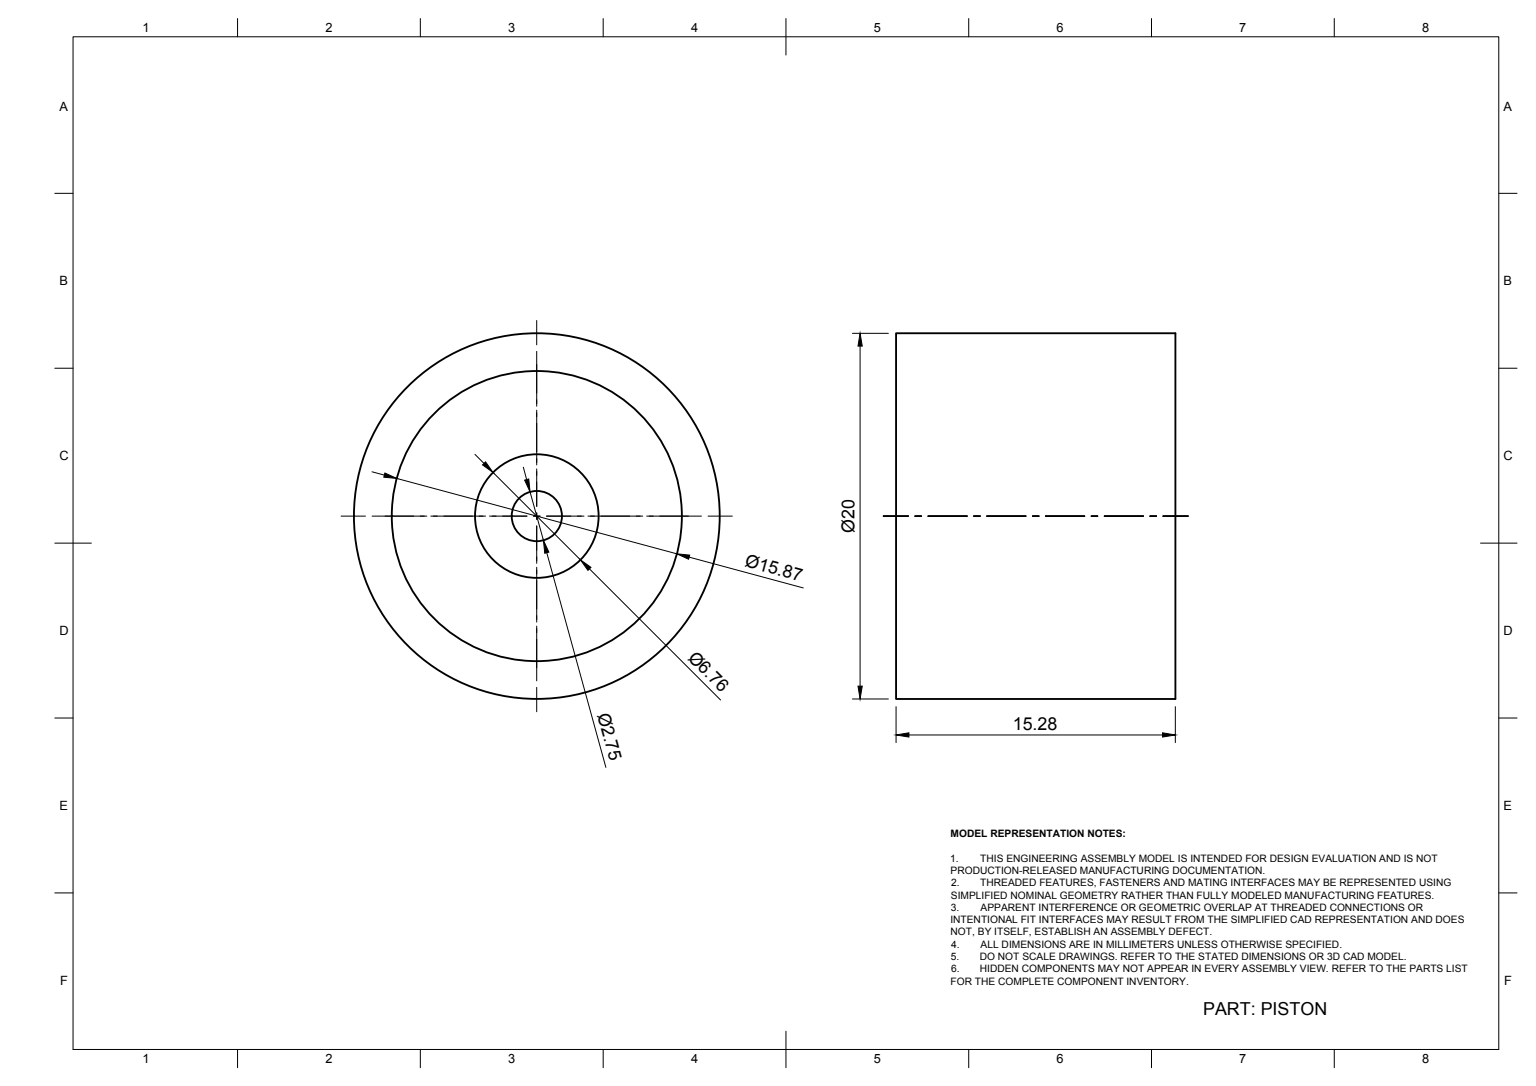
ISO-10303-21;
HEADER;
/* Generated by software containing ST-Developer
 * from STEP Tools, Inc. (www.steptools.com) 
 */

FILE_DESCRIPTION(
/* description */ (''),
/* implementation_level */ '2;1');

FILE_NAME(
/* name */ 'Piston.step',
/* time_stamp */ '2026-10-04T22:56:18-07:00',
/* author */ (''),
/* organization */ (''),
/* preprocessor_version */ 'ST-DEVELOPER v20.2',
/* originating_system */ 'Autodesk Translation Framework v15.15.0.0',
/* authorisation */ '');

FILE_SCHEMA (('AUTOMOTIVE_DESIGN { 1 0 10303 214 3 1 1 }'));
ENDSEC;

DATA;
#10=MECHANICAL_DESIGN_GEOMETRIC_PRESENTATION_REPRESENTATION('',(#191),#14544);
#171=TOROIDAL_SURFACE('',#1951,2.67974687627927,0.7);
#175=SHAPE_REPRESENTATION_RELATIONSHIP('SRR','None',#14577,#183);
#183=ADVANCED_BREP_SHAPE_REPRESENTATION('',(#199),#14537);
#191=STYLED_ITEM('',(#14626),#199);
#199=MANIFOLD_SOLID_BREP('Body1',#1827);
#208=LINE('',#2618,#264);
#209=LINE('',#2625,#265);
#210=LINE('',#2632,#266);
#211=LINE('',#2639,#267);
#212=LINE('',#2650,#268);
#213=LINE('',#2657,#269);
#214=LINE('',#2664,#270);
#264=VECTOR('',#2160,10.0021025234003);
#265=VECTOR('',#2169,7.93438181172474);
#266=VECTOR('',#2178,2.72924949802694);
#267=VECTOR('',#2187,3.37974687627927);
#268=VECTOR('',#2202,1.37433660530134);
#269=VECTOR('',#2211,2.58871463782345);
#270=VECTOR('',#2222,1.25945989284257);
#320=CYLINDRICAL_SURFACE('',#1936,10.0021025234003);
#321=CYLINDRICAL_SURFACE('',#1941,7.93438181172474);
#322=CYLINDRICAL_SURFACE('',#1945,2.72924949802694);
#323=CYLINDRICAL_SURFACE('',#1949,3.37974687627927);
#324=CYLINDRICAL_SURFACE('',#1956,1.37433660530134);
#325=CYLINDRICAL_SURFACE('',#1960,2.58871463782345);
#326=CYLINDRICAL_SURFACE('',#1965,1.25945989284257);
#372=FACE_BOUND('',#513,.T.);
#373=FACE_BOUND('',#516,.T.);
#374=FACE_BOUND('',#519,.T.);
#375=FACE_BOUND('',#523,.T.);
#376=FACE_BOUND('',#526,.T.);
#377=FACE_BOUND('',#530,.T.);
#403=FACE_OUTER_BOUND('',#510,.T.);
#404=FACE_OUTER_BOUND('',#511,.T.);
#405=FACE_OUTER_BOUND('',#512,.T.);
#406=FACE_OUTER_BOUND('',#514,.T.);
#407=FACE_OUTER_BOUND('',#515,.T.);
#408=FACE_OUTER_BOUND('',#517,.T.);
#409=FACE_OUTER_BOUND('',#518,.T.);
#410=FACE_OUTER_BOUND('',#520,.T.);
#411=FACE_OUTER_BOUND('',#521,.T.);
#412=FACE_OUTER_BOUND('',#522,.T.);
#413=FACE_OUTER_BOUND('',#524,.T.);
#414=FACE_OUTER_BOUND('',#525,.T.);
#415=FACE_OUTER_BOUND('',#527,.T.);
#416=FACE_OUTER_BOUND('',#528,.T.);
#417=FACE_OUTER_BOUND('',#529,.T.);
#418=FACE_OUTER_BOUND('',#531,.T.);
#510=EDGE_LOOP('',(#1183));
#511=EDGE_LOOP('',(#1184,#1185,#1186,#1187));
#512=EDGE_LOOP('',(#1188));
#513=EDGE_LOOP('',(#1189));
#514=EDGE_LOOP('',(#1190,#1191,#1192,#1193));
#515=EDGE_LOOP('',(#1194));
#516=EDGE_LOOP('',(#1195));
#517=EDGE_LOOP('',(#1196,#1197,#1198,#1199));
#518=EDGE_LOOP('',(#1200));
#519=EDGE_LOOP('',(#1201));
#520=EDGE_LOOP('',(#1202,#1203,#1204,#1205));
#521=EDGE_LOOP('',(#1206,#1207,#1208,#1209));
#522=EDGE_LOOP('',(#1210));
#523=EDGE_LOOP('',(#1211));
#524=EDGE_LOOP('',(#1212,#1213,#1214,#1215));
#525=EDGE_LOOP('',(#1216));
#526=EDGE_LOOP('',(#1217));
#527=EDGE_LOOP('',(#1218,#1219,#1220,#1221));
#528=EDGE_LOOP('',(#1222));
#529=EDGE_LOOP('',(#1223));
#530=EDGE_LOOP('',(#1224));
#531=EDGE_LOOP('',(#1225,#1226,#1227,#1228));
#642=CIRCLE('',#1935,1.25945989284257);
#643=CIRCLE('',#1937,10.0021025234003);
#644=CIRCLE('',#1938,10.0021025234003);
#645=CIRCLE('',#1940,7.93438181172474);
#646=CIRCLE('',#1942,7.93438181172474);
#647=CIRCLE('',#1944,2.72924949802694);
#648=CIRCLE('',#1946,2.72924949802694);
#649=CIRCLE('',#1948,3.37974687627927);
#650=CIRCLE('',#1950,3.37974687627927);
#651=CIRCLE('',#1952,0.7);
#652=CIRCLE('',#1953,2.67974687627927);
#653=CIRCLE('',#1955,1.37433660530134);
#654=CIRCLE('',#1957,1.37433660530134);
#655=CIRCLE('',#1959,2.58871463782345);
#656=CIRCLE('',#1961,2.58871463782345);
#657=CIRCLE('',#1964,1.25945989284257);
#729=VERTEX_POINT('',#2612);
#730=VERTEX_POINT('',#2615);
#731=VERTEX_POINT('',#2617);
#732=VERTEX_POINT('',#2621);
#733=VERTEX_POINT('',#2624);
#734=VERTEX_POINT('',#2628);
#735=VERTEX_POINT('',#2631);
#736=VERTEX_POINT('',#2635);
#737=VERTEX_POINT('',#2638);
#738=VERTEX_POINT('',#2642);
#739=VERTEX_POINT('',#2646);
#740=VERTEX_POINT('',#2649);
#741=VERTEX_POINT('',#2653);
#742=VERTEX_POINT('',#2656);
#743=VERTEX_POINT('',#2661);
#920=EDGE_CURVE('',#729,#729,#642,.T.);
#921=EDGE_CURVE('',#730,#730,#643,.T.);
#922=EDGE_CURVE('',#730,#731,#208,.T.);
#923=EDGE_CURVE('',#731,#731,#644,.T.);
#924=EDGE_CURVE('',#732,#732,#645,.T.);
#925=EDGE_CURVE('',#732,#733,#209,.T.);
#926=EDGE_CURVE('',#733,#733,#646,.T.);
#927=EDGE_CURVE('',#734,#734,#647,.T.);
#928=EDGE_CURVE('',#734,#735,#210,.T.);
#929=EDGE_CURVE('',#735,#735,#648,.T.);
#930=EDGE_CURVE('',#736,#736,#649,.T.);
#931=EDGE_CURVE('',#736,#737,#211,.T.);
#932=EDGE_CURVE('',#737,#737,#650,.T.);
#933=EDGE_CURVE('',#737,#738,#651,.T.);
#934=EDGE_CURVE('',#738,#738,#652,.T.);
#935=EDGE_CURVE('',#739,#739,#653,.T.);
#936=EDGE_CURVE('',#739,#740,#212,.T.);
#937=EDGE_CURVE('',#740,#740,#654,.T.);
#938=EDGE_CURVE('',#741,#741,#655,.T.);
#939=EDGE_CURVE('',#741,#742,#213,.T.);
#940=EDGE_CURVE('',#742,#742,#656,.T.);
#941=EDGE_CURVE('',#743,#743,#657,.T.);
#942=EDGE_CURVE('',#729,#743,#214,.T.);
#1183=ORIENTED_EDGE('',*,*,#920,.T.);
#1184=ORIENTED_EDGE('',*,*,#921,.F.);
#1185=ORIENTED_EDGE('',*,*,#922,.T.);
#1186=ORIENTED_EDGE('',*,*,#923,.T.);
#1187=ORIENTED_EDGE('',*,*,#922,.F.);
#1188=ORIENTED_EDGE('',*,*,#923,.F.);
#1189=ORIENTED_EDGE('',*,*,#924,.T.);
#1190=ORIENTED_EDGE('',*,*,#924,.F.);
#1191=ORIENTED_EDGE('',*,*,#925,.T.);
#1192=ORIENTED_EDGE('',*,*,#926,.T.);
#1193=ORIENTED_EDGE('',*,*,#925,.F.);
#1194=ORIENTED_EDGE('',*,*,#926,.F.);
#1195=ORIENTED_EDGE('',*,*,#927,.T.);
#1196=ORIENTED_EDGE('',*,*,#927,.F.);
#1197=ORIENTED_EDGE('',*,*,#928,.T.);
#1198=ORIENTED_EDGE('',*,*,#929,.T.);
#1199=ORIENTED_EDGE('',*,*,#928,.F.);
#1200=ORIENTED_EDGE('',*,*,#930,.T.);
#1201=ORIENTED_EDGE('',*,*,#929,.F.);
#1202=ORIENTED_EDGE('',*,*,#930,.F.);
#1203=ORIENTED_EDGE('',*,*,#931,.T.);
#1204=ORIENTED_EDGE('',*,*,#932,.T.);
#1205=ORIENTED_EDGE('',*,*,#931,.F.);
#1206=ORIENTED_EDGE('',*,*,#932,.F.);
#1207=ORIENTED_EDGE('',*,*,#933,.T.);
#1208=ORIENTED_EDGE('',*,*,#934,.T.);
#1209=ORIENTED_EDGE('',*,*,#933,.F.);
#1210=ORIENTED_EDGE('',*,*,#934,.F.);
#1211=ORIENTED_EDGE('',*,*,#935,.T.);
#1212=ORIENTED_EDGE('',*,*,#935,.F.);
#1213=ORIENTED_EDGE('',*,*,#936,.T.);
#1214=ORIENTED_EDGE('',*,*,#937,.T.);
#1215=ORIENTED_EDGE('',*,*,#936,.F.);
#1216=ORIENTED_EDGE('',*,*,#938,.T.);
#1217=ORIENTED_EDGE('',*,*,#937,.F.);
#1218=ORIENTED_EDGE('',*,*,#938,.F.);
#1219=ORIENTED_EDGE('',*,*,#939,.T.);
#1220=ORIENTED_EDGE('',*,*,#940,.T.);
#1221=ORIENTED_EDGE('',*,*,#939,.F.);
#1222=ORIENTED_EDGE('',*,*,#940,.F.);
#1223=ORIENTED_EDGE('',*,*,#921,.T.);
#1224=ORIENTED_EDGE('',*,*,#941,.T.);
#1225=ORIENTED_EDGE('',*,*,#920,.F.);
#1226=ORIENTED_EDGE('',*,*,#942,.T.);
#1227=ORIENTED_EDGE('',*,*,#941,.F.);
#1228=ORIENTED_EDGE('',*,*,#942,.F.);
#1687=PLANE('',#1934);
#1688=PLANE('',#1939);
#1689=PLANE('',#1943);
#1690=PLANE('',#1947);
#1691=PLANE('',#1954);
#1692=PLANE('',#1958);
#1693=PLANE('',#1962);
#1694=PLANE('',#1963);
#1725=ADVANCED_FACE('',(#403),#1687,.T.);
#1726=ADVANCED_FACE('',(#404),#320,.T.);
#1727=ADVANCED_FACE('',(#405,#372),#1688,.T.);
#1728=ADVANCED_FACE('',(#406),#321,.F.);
#1729=ADVANCED_FACE('',(#407,#373),#1689,.T.);
#1730=ADVANCED_FACE('',(#408),#322,.T.);
#1731=ADVANCED_FACE('',(#409,#374),#1690,.T.);
#1732=ADVANCED_FACE('',(#410),#323,.T.);
#1733=ADVANCED_FACE('',(#411),#171,.T.);
#1734=ADVANCED_FACE('',(#412,#375),#1691,.T.);
#1735=ADVANCED_FACE('',(#413),#324,.F.);
#1736=ADVANCED_FACE('',(#414,#376),#1692,.T.);
#1737=ADVANCED_FACE('',(#415),#325,.F.);
#1738=ADVANCED_FACE('',(#416),#1693,.T.);
#1739=ADVANCED_FACE('',(#417,#377),#1694,.F.);
#1740=ADVANCED_FACE('',(#418),#326,.F.);
#1827=CLOSED_SHELL('',(#1725,#1726,#1727,#1728,#1729,#1730,#1731,#1732,
#1733,#1734,#1735,#1736,#1737,#1738,#1739,#1740));
#1933=AXIS2_PLACEMENT_3D('',#2610,#2150,#2151);
#1934=AXIS2_PLACEMENT_3D('',#2611,#2152,#2153);
#1935=AXIS2_PLACEMENT_3D('',#2613,#2154,#2155);
#1936=AXIS2_PLACEMENT_3D('',#2614,#2156,#2157);
#1937=AXIS2_PLACEMENT_3D('',#2616,#2158,#2159);
#1938=AXIS2_PLACEMENT_3D('',#2619,#2161,#2162);
#1939=AXIS2_PLACEMENT_3D('',#2620,#2163,#2164);
#1940=AXIS2_PLACEMENT_3D('',#2622,#2165,#2166);
#1941=AXIS2_PLACEMENT_3D('',#2623,#2167,#2168);
#1942=AXIS2_PLACEMENT_3D('',#2626,#2170,#2171);
#1943=AXIS2_PLACEMENT_3D('',#2627,#2172,#2173);
#1944=AXIS2_PLACEMENT_3D('',#2629,#2174,#2175);
#1945=AXIS2_PLACEMENT_3D('',#2630,#2176,#2177);
#1946=AXIS2_PLACEMENT_3D('',#2633,#2179,#2180);
#1947=AXIS2_PLACEMENT_3D('',#2634,#2181,#2182);
#1948=AXIS2_PLACEMENT_3D('',#2636,#2183,#2184);
#1949=AXIS2_PLACEMENT_3D('',#2637,#2185,#2186);
#1950=AXIS2_PLACEMENT_3D('',#2640,#2188,#2189);
#1951=AXIS2_PLACEMENT_3D('',#2641,#2190,#2191);
#1952=AXIS2_PLACEMENT_3D('',#2643,#2192,#2193);
#1953=AXIS2_PLACEMENT_3D('',#2644,#2194,#2195);
#1954=AXIS2_PLACEMENT_3D('',#2645,#2196,#2197);
#1955=AXIS2_PLACEMENT_3D('',#2647,#2198,#2199);
#1956=AXIS2_PLACEMENT_3D('',#2648,#2200,#2201);
#1957=AXIS2_PLACEMENT_3D('',#2651,#2203,#2204);
#1958=AXIS2_PLACEMENT_3D('',#2652,#2205,#2206);
#1959=AXIS2_PLACEMENT_3D('',#2654,#2207,#2208);
#1960=AXIS2_PLACEMENT_3D('',#2655,#2209,#2210);
#1961=AXIS2_PLACEMENT_3D('',#2658,#2212,#2213);
#1962=AXIS2_PLACEMENT_3D('',#2659,#2214,#2215);
#1963=AXIS2_PLACEMENT_3D('',#2660,#2216,#2217);
#1964=AXIS2_PLACEMENT_3D('',#2662,#2218,#2219);
#1965=AXIS2_PLACEMENT_3D('',#2663,#2220,#2221);
#2150=DIRECTION('axis',(0.,0.,1.));
#2151=DIRECTION('refdir',(1.,0.,0.));
#2152=DIRECTION('center_axis',(0.,0.,1.));
#2153=DIRECTION('ref_axis',(1.,0.,0.));
#2154=DIRECTION('center_axis',(0.,0.,1.));
#2155=DIRECTION('ref_axis',(1.,0.,0.));
#2156=DIRECTION('center_axis',(0.,0.,1.));
#2157=DIRECTION('ref_axis',(1.,0.,0.));
#2158=DIRECTION('center_axis',(0.,0.,1.));
#2159=DIRECTION('ref_axis',(1.,0.,0.));
#2160=DIRECTION('',(0.,0.,-1.));
#2161=DIRECTION('center_axis',(0.,0.,1.));
#2162=DIRECTION('ref_axis',(1.,0.,0.));
#2163=DIRECTION('center_axis',(0.,0.,-1.));
#2164=DIRECTION('ref_axis',(-1.,0.,0.));
#2165=DIRECTION('center_axis',(0.,0.,1.));
#2166=DIRECTION('ref_axis',(1.,0.,0.));
#2167=DIRECTION('center_axis',(0.,0.,1.));
#2168=DIRECTION('ref_axis',(1.,0.,0.));
#2169=DIRECTION('',(0.,0.,1.));
#2170=DIRECTION('center_axis',(0.,0.,1.));
#2171=DIRECTION('ref_axis',(1.,0.,0.));
#2172=DIRECTION('center_axis',(0.,0.,-1.));
#2173=DIRECTION('ref_axis',(-1.,0.,0.));
#2174=DIRECTION('center_axis',(0.,0.,1.));
#2175=DIRECTION('ref_axis',(1.,0.,0.));
#2176=DIRECTION('center_axis',(0.,0.,1.));
#2177=DIRECTION('ref_axis',(1.,0.,0.));
#2178=DIRECTION('',(0.,0.,-1.));
#2179=DIRECTION('center_axis',(0.,0.,1.));
#2180=DIRECTION('ref_axis',(1.,0.,0.));
#2181=DIRECTION('center_axis',(0.,0.,1.));
#2182=DIRECTION('ref_axis',(1.,0.,0.));
#2183=DIRECTION('center_axis',(0.,0.,1.));
#2184=DIRECTION('ref_axis',(1.,0.,0.));
#2185=DIRECTION('center_axis',(0.,0.,1.));
#2186=DIRECTION('ref_axis',(1.,0.,0.));
#2187=DIRECTION('',(0.,0.,-1.));
#2188=DIRECTION('center_axis',(0.,0.,1.));
#2189=DIRECTION('ref_axis',(1.,0.,0.));
#2190=DIRECTION('center_axis',(0.,0.,1.));
#2191=DIRECTION('ref_axis',(1.,0.,0.));
#2192=DIRECTION('center_axis',(1.22464679914735E-16,-1.,0.));
#2193=DIRECTION('ref_axis',(-1.,-1.22464679914735E-16,0.));
#2194=DIRECTION('center_axis',(0.,0.,1.));
#2195=DIRECTION('ref_axis',(1.,0.,0.));
#2196=DIRECTION('center_axis',(0.,0.,-1.));
#2197=DIRECTION('ref_axis',(-1.,0.,0.));
#2198=DIRECTION('center_axis',(0.,0.,1.));
#2199=DIRECTION('ref_axis',(1.,0.,0.));
#2200=DIRECTION('center_axis',(0.,0.,1.));
#2201=DIRECTION('ref_axis',(1.,0.,0.));
#2202=DIRECTION('',(0.,0.,1.));
#2203=DIRECTION('center_axis',(0.,0.,1.));
#2204=DIRECTION('ref_axis',(1.,0.,0.));
#2205=DIRECTION('center_axis',(0.,0.,1.));
#2206=DIRECTION('ref_axis',(1.,0.,0.));
#2207=DIRECTION('center_axis',(0.,0.,1.));
#2208=DIRECTION('ref_axis',(1.,0.,0.));
#2209=DIRECTION('center_axis',(0.,0.,1.));
#2210=DIRECTION('ref_axis',(1.,0.,0.));
#2211=DIRECTION('',(0.,0.,1.));
#2212=DIRECTION('center_axis',(0.,0.,1.));
#2213=DIRECTION('ref_axis',(1.,0.,0.));
#2214=DIRECTION('center_axis',(0.,0.,-1.));
#2215=DIRECTION('ref_axis',(-1.,0.,0.));
#2216=DIRECTION('center_axis',(0.,0.,-1.));
#2217=DIRECTION('ref_axis',(-1.,0.,0.));
#2218=DIRECTION('center_axis',(0.,0.,-1.));
#2219=DIRECTION('ref_axis',(1.,0.,0.));
#2220=DIRECTION('center_axis',(0.,0.,1.));
#2221=DIRECTION('ref_axis',(1.,0.,0.));
#2222=DIRECTION('',(0.,0.,1.));
#2610=CARTESIAN_POINT('',(0.,0.,0.));
#2611=CARTESIAN_POINT('Origin',(0.,0.,58.1431215754561));
#2612=CARTESIAN_POINT('',(-1.25945989284257,-1.54239352642412E-16,58.1431215754561));
#2613=CARTESIAN_POINT('Origin',(0.,0.,58.1431215754561));
#2614=CARTESIAN_POINT('Origin',(0.,0.,53.7053570659329));
#2615=CARTESIAN_POINT('',(-10.0021025234003,-1.22490428400259E-15,61.3445102174369));
#2616=CARTESIAN_POINT('Origin',(0.,0.,61.3445102174369));
#2617=CARTESIAN_POINT('',(-10.0021025234003,-1.22490428400259E-15,46.0662039144288));
#2618=CARTESIAN_POINT('',(-10.0021025234003,-1.22490428400258E-15,53.7053570659329));
#2619=CARTESIAN_POINT('Origin',(0.,0.,46.0662039144288));
#2620=CARTESIAN_POINT('Origin',(10.0021025234003,0.,46.0662039144288));
#2621=CARTESIAN_POINT('',(-7.93438181172474,-9.71681528894168E-16,46.0662039144288));
#2622=CARTESIAN_POINT('Origin',(0.,0.,46.0662039144288));
#2623=CARTESIAN_POINT('Origin',(0.,0.,52.1046627449425));
#2624=CARTESIAN_POINT('',(-7.93438181172474,-9.71681528894168E-16,58.1431215754561));
#2625=CARTESIAN_POINT('',(-7.93438181172474,-9.71681528894168E-16,52.1046627449425));
#2626=CARTESIAN_POINT('Origin',(0.,0.,58.1431215754561));
#2627=CARTESIAN_POINT('Origin',(7.93438181172474,0.,58.1431215754561));
#2628=CARTESIAN_POINT('',(-2.72924949802694,-3.34236666183321E-16,58.1431215754561));
#2629=CARTESIAN_POINT('Origin',(0.,0.,58.1431215754561));
#2630=CARTESIAN_POINT('Origin',(0.,0.,57.7133622810548));
#2631=CARTESIAN_POINT('',(-2.72924949802694,-3.34236666183321E-16,57.2836029866534));
#2632=CARTESIAN_POINT('',(-2.72924949802694,-3.34236666183321E-16,57.7133622810548));
#2633=CARTESIAN_POINT('Origin',(0.,0.,57.2836029866534));
#2634=CARTESIAN_POINT('Origin',(2.72924949802694,0.,57.2836029866534));
#2635=CARTESIAN_POINT('',(-3.37974687627927,-4.13899619396367E-16,57.2836029866534));
#2636=CARTESIAN_POINT('Origin',(0.,0.,57.2836029866534));
#2637=CARTESIAN_POINT('Origin',(0.,0.,53.9082407428739));
#2638=CARTESIAN_POINT('',(-3.37974687627927,-4.13899619396367E-16,50.5328784990943));
#2639=CARTESIAN_POINT('',(-3.37974687627927,-4.13899619396367E-16,53.9082407428739));
#2640=CARTESIAN_POINT('Origin',(0.,0.,50.5328784990943));
#2641=CARTESIAN_POINT('Origin',(0.,0.,50.5328784990943));
#2642=CARTESIAN_POINT('',(-2.67974687627927,-3.28174343456053E-16,49.8328784990943));
#2643=CARTESIAN_POINT('Origin',(-2.67974687627927,-3.28174343456053E-16,
50.5328784990943));
#2644=CARTESIAN_POINT('Origin',(0.,0.,49.8328784990943));
#2645=CARTESIAN_POINT('Origin',(2.67974687627927,0.,49.8328784990943));
#2646=CARTESIAN_POINT('',(-1.37433660530134,-1.68307692463333E-16,49.8328784990943));
#2647=CARTESIAN_POINT('Origin',(0.,0.,49.8328784990943));
#2648=CARTESIAN_POINT('Origin',(0.,0.,50.0785885840682));
#2649=CARTESIAN_POINT('',(-1.37433660530134,-1.68307692463333E-16,50.3242986690421));
#2650=CARTESIAN_POINT('',(-1.37433660530134,-1.68307692463333E-16,50.0785885840682));
#2651=CARTESIAN_POINT('Origin',(0.,0.,50.3242986690421));
#2652=CARTESIAN_POINT('Origin',(1.37433660530134,0.,50.3242986690421));
#2653=CARTESIAN_POINT('',(-2.58871463782345,-3.17026109511639E-16,50.3242986690421));
#2654=CARTESIAN_POINT('Origin',(0.,0.,50.3242986690421));
#2655=CARTESIAN_POINT('Origin',(0.,0.,53.0505398104803));
#2656=CARTESIAN_POINT('',(-2.58871463782345,-3.17026109511639E-16,55.7767809519186));
#2657=CARTESIAN_POINT('',(-2.58871463782345,-3.17026109511639E-16,53.0505398104803));
#2658=CARTESIAN_POINT('Origin',(0.,0.,55.7767809519186));
#2659=CARTESIAN_POINT('Origin',(2.58871463782345,0.,55.7767809519186));
#2660=CARTESIAN_POINT('Origin',(10.0021025234003,0.,61.3445102174369));
#2661=CARTESIAN_POINT('',(-1.25945989284257,1.54239352642412E-16,61.3445102174369));
#2662=CARTESIAN_POINT('Origin',(0.,0.,61.3445102174369));
#2663=CARTESIAN_POINT('Origin',(0.,0.,60.205945294667));
#2664=CARTESIAN_POINT('',(-1.25945989284257,-1.54239352642412E-16,60.205945294667));
#14527=UNCERTAINTY_MEASURE_WITH_UNIT(LENGTH_MEASURE(0.01),#14545,
'DISTANCE_ACCURACY_VALUE',
'Maximum model space distance between geometric entities at asserted c
onnectivities');
#14534=UNCERTAINTY_MEASURE_WITH_UNIT(LENGTH_MEASURE(0.01),#14545,
'DISTANCE_ACCURACY_VALUE',
'Maximum model space distance between geometric entities at asserted c
onnectivities');
#14537=(
GEOMETRIC_REPRESENTATION_CONTEXT(3)
GLOBAL_UNCERTAINTY_ASSIGNED_CONTEXT((#14527))
GLOBAL_UNIT_ASSIGNED_CONTEXT((#14545,#14547,#14548))
REPRESENTATION_CONTEXT('','3D')
);
#14544=(
GEOMETRIC_REPRESENTATION_CONTEXT(3)
GLOBAL_UNCERTAINTY_ASSIGNED_CONTEXT((#14534))
GLOBAL_UNIT_ASSIGNED_CONTEXT((#14545,#14547,#14548))
REPRESENTATION_CONTEXT('','3D')
);
#14545=(
LENGTH_UNIT()
NAMED_UNIT(*)
SI_UNIT(.MILLI.,.METRE.)
);
#14547=(
NAMED_UNIT(*)
PLANE_ANGLE_UNIT()
SI_UNIT($,.RADIAN.)
);
#14548=(
NAMED_UNIT(*)
SI_UNIT($,.STERADIAN.)
SOLID_ANGLE_UNIT()
);
#14551=SHAPE_DEFINITION_REPRESENTATION(#14560,#14577);
#14560=PRODUCT_DEFINITION_SHAPE('',$,#14587);
#14577=SHAPE_REPRESENTATION('',(#1933),#14537);
#14584=PRODUCT_DEFINITION_CONTEXT('part definition',#14613,'design');
#14587=PRODUCT_DEFINITION('Piston','Piston',#14596,#14584);
#14596=PRODUCT_DEFINITION_FORMATION('',$,#14617);
#14613=APPLICATION_CONTEXT(
'Core Data for Automotive Mechanical Design Process');
#14614=PRODUCT_CONTEXT('part definition',#14613,'mechanical');
#14617=PRODUCT('Piston','Piston',$,(#14614));
#14626=PRESENTATION_STYLE_ASSIGNMENT((#14630));
#14630=SURFACE_STYLE_USAGE(.BOTH.,#14634);
#14634=SURFACE_SIDE_STYLE('',(#14638));
#14638=SURFACE_STYLE_FILL_AREA(#14642);
#14642=FILL_AREA_STYLE('Opaque(39,39,39)',(#14646));
#14646=FILL_AREA_STYLE_COLOUR('Opaque(39,39,39)',#14650);
#14650=COLOUR_RGB('Opaque(39,39,39)', 0.66274510, 0.83137255, 0.94901961);
ENDSEC;
END-ISO-10303-21;
